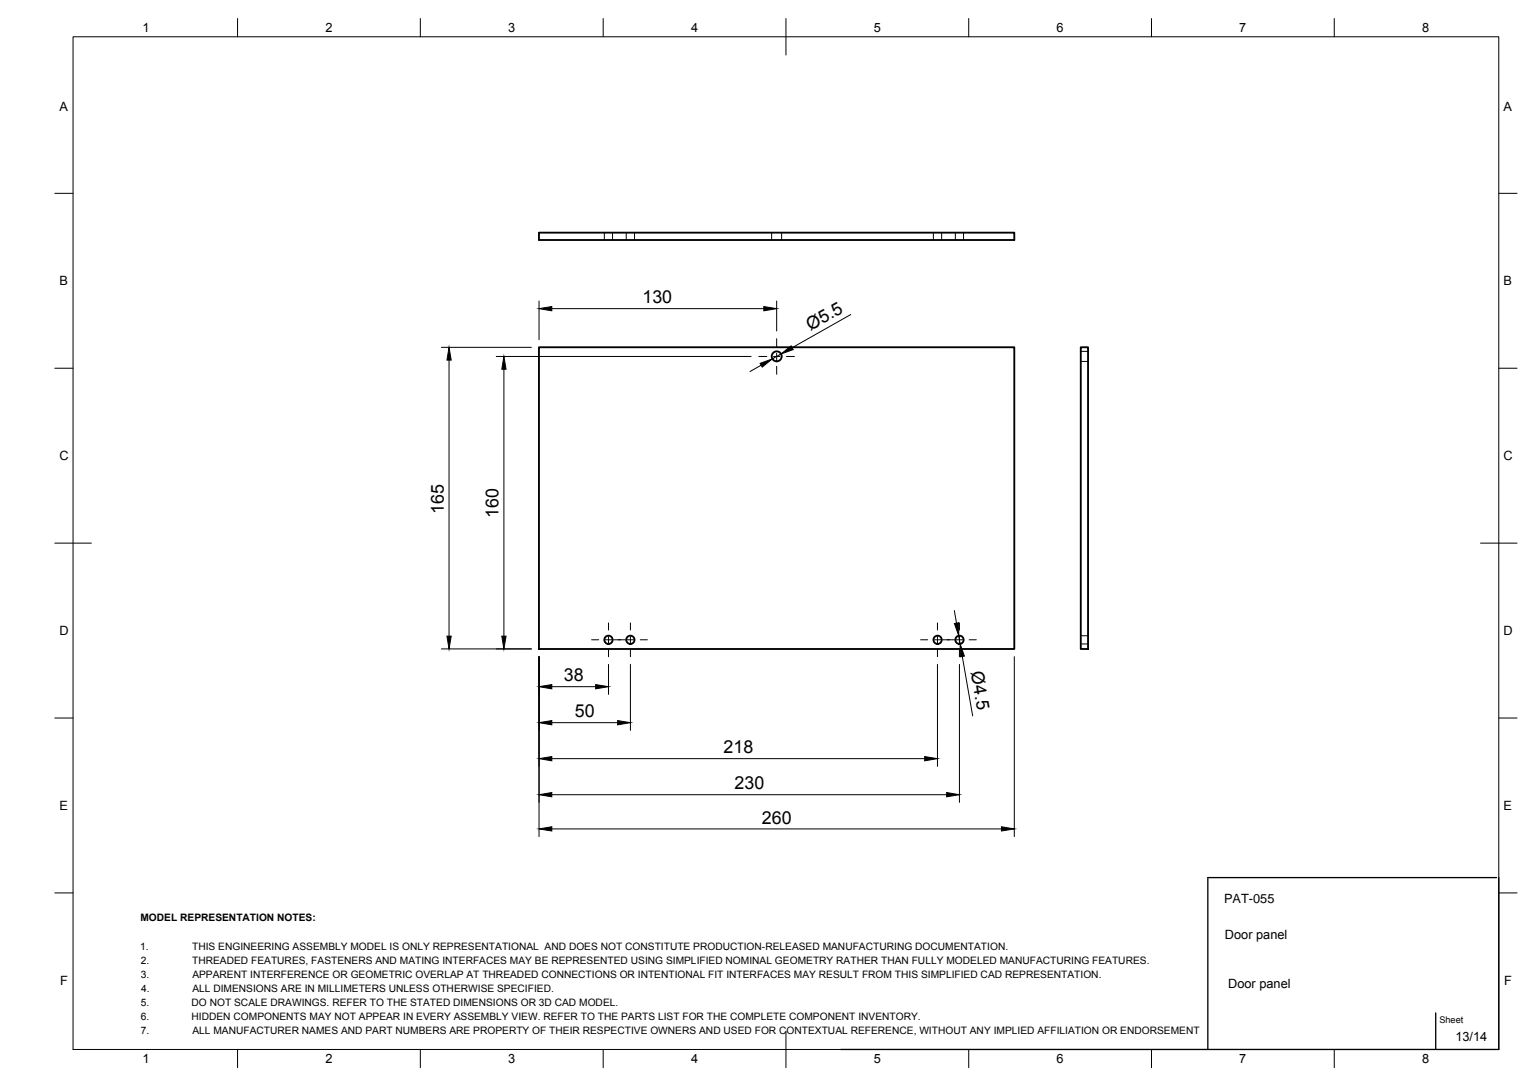
ISO-10303-21;
HEADER;
/* Generated by software containing ST-Developer
 * from STEP Tools, Inc. (www.steptools.com) 
 */

FILE_DESCRIPTION(
/* description */ ('Hinged panel with latch'),
/* implementation_level */ '2;1');

FILE_NAME(
/* name */ 'Door panel.step',
/* time_stamp */ '2026-10-27T20:36:01-07:00',
/* author */ (''),
/* organization */ (''),
/* preprocessor_version */ 'ST-DEVELOPER v20.2',
/* originating_system */ 'Autodesk Translation Framework v15.17.0.0',
/* authorisation */ '');

FILE_SCHEMA (('AUTOMOTIVE_DESIGN { 1 0 10303 214 3 1 1 }'));
ENDSEC;

DATA;
#10=MECHANICAL_DESIGN_GEOMETRIC_PRESENTATION_REPRESENTATION('',(#304),#6743);
#272=SHAPE_REPRESENTATION_RELATIONSHIP('SRR','None',#6848,#288);
#288=ADVANCED_BREP_SHAPE_REPRESENTATION('',(#319),#6734);
#304=STYLED_ITEM('',(#6989),#319);
#319=MANIFOLD_SOLID_BREP('Body1',#3807);
#346=FACE_BOUND('',#870,.T.);
#347=FACE_BOUND('',#871,.T.);
#348=FACE_BOUND('',#872,.T.);
#349=FACE_BOUND('',#873,.T.);
#350=FACE_BOUND('',#874,.T.);
#351=FACE_BOUND('',#877,.T.);
#352=FACE_BOUND('',#878,.T.);
#353=FACE_BOUND('',#879,.T.);
#354=FACE_BOUND('',#880,.T.);
#355=FACE_BOUND('',#881,.T.);
#462=PLANE('',#4181);
#463=PLANE('',#4182);
#464=PLANE('',#4183);
#465=PLANE('',#4184);
#466=PLANE('',#4185);
#467=PLANE('',#4186);
#637=FACE_OUTER_BOUND('',#864,.T.);
#638=FACE_OUTER_BOUND('',#865,.T.);
#639=FACE_OUTER_BOUND('',#866,.T.);
#640=FACE_OUTER_BOUND('',#867,.T.);
#641=FACE_OUTER_BOUND('',#868,.T.);
#642=FACE_OUTER_BOUND('',#869,.T.);
#643=FACE_OUTER_BOUND('',#875,.T.);
#644=FACE_OUTER_BOUND('',#876,.T.);
#645=FACE_OUTER_BOUND('',#882,.T.);
#646=FACE_OUTER_BOUND('',#883,.T.);
#647=FACE_OUTER_BOUND('',#884,.T.);
#864=EDGE_LOOP('',(#3162,#3163,#3164,#3165));
#865=EDGE_LOOP('',(#3166,#3167,#3168,#3169));
#866=EDGE_LOOP('',(#3170,#3171,#3172,#3173));
#867=EDGE_LOOP('',(#3174,#3175,#3176,#3177));
#868=EDGE_LOOP('',(#3178,#3179,#3180,#3181));
#869=EDGE_LOOP('',(#3182,#3183,#3184,#3185));
#870=EDGE_LOOP('',(#3186));
#871=EDGE_LOOP('',(#3187));
#872=EDGE_LOOP('',(#3188));
#873=EDGE_LOOP('',(#3189));
#874=EDGE_LOOP('',(#3190));
#875=EDGE_LOOP('',(#3191,#3192,#3193,#3194));
#876=EDGE_LOOP('',(#3195,#3196,#3197,#3198));
#877=EDGE_LOOP('',(#3199));
#878=EDGE_LOOP('',(#3200));
#879=EDGE_LOOP('',(#3201));
#880=EDGE_LOOP('',(#3202));
#881=EDGE_LOOP('',(#3203));
#882=EDGE_LOOP('',(#3204,#3205,#3206,#3207));
#883=EDGE_LOOP('',(#3208,#3209,#3210,#3211));
#884=EDGE_LOOP('',(#3212,#3213,#3214,#3215));
#1216=LINE('',#6185,#1574);
#1217=LINE('',#6191,#1575);
#1218=LINE('',#6197,#1576);
#1219=LINE('',#6203,#1577);
#1220=LINE('',#6209,#1578);
#1221=LINE('',#6214,#1579);
#1222=LINE('',#6216,#1580);
#1223=LINE('',#6218,#1581);
#1224=LINE('',#6219,#1582);
#1225=LINE('',#6222,#1583);
#1226=LINE('',#6224,#1584);
#1227=LINE('',#6225,#1585);
#1228=LINE('',#6228,#1586);
#1229=LINE('',#6230,#1587);
#1230=LINE('',#6231,#1588);
#1231=LINE('',#6233,#1589);
#1232=LINE('',#6234,#1590);
#1574=VECTOR('',#4946,0.274999999999999);
#1575=VECTOR('',#4953,0.225);
#1576=VECTOR('',#4960,0.225);
#1577=VECTOR('',#4967,0.225);
#1578=VECTOR('',#4974,0.225);
#1579=VECTOR('',#4979,1.);
#1580=VECTOR('',#4980,1.);
#1581=VECTOR('',#4981,1.);
#1582=VECTOR('',#4982,1.);
#1583=VECTOR('',#4985,1.);
#1584=VECTOR('',#4986,1.);
#1585=VECTOR('',#4987,1.);
#1586=VECTOR('',#4990,1.);
#1587=VECTOR('',#4991,1.);
#1588=VECTOR('',#4992,1.);
#1589=VECTOR('',#4995,1.);
#1590=VECTOR('',#4996,1.);
#1742=CIRCLE('',#4167,0.274999999999999);
#1743=CIRCLE('',#4168,0.274999999999999);
#1744=CIRCLE('',#4170,0.225);
#1745=CIRCLE('',#4171,0.225);
#1746=CIRCLE('',#4173,0.225);
#1747=CIRCLE('',#4174,0.225);
#1748=CIRCLE('',#4176,0.225);
#1749=CIRCLE('',#4177,0.225);
#1750=CIRCLE('',#4179,0.225);
#1751=CIRCLE('',#4180,0.225);
#1980=VERTEX_POINT('',#6182);
#1981=VERTEX_POINT('',#6184);
#1982=VERTEX_POINT('',#6188);
#1983=VERTEX_POINT('',#6190);
#1984=VERTEX_POINT('',#6194);
#1985=VERTEX_POINT('',#6196);
#1986=VERTEX_POINT('',#6200);
#1987=VERTEX_POINT('',#6202);
#1988=VERTEX_POINT('',#6206);
#1989=VERTEX_POINT('',#6208);
#1990=VERTEX_POINT('',#6212);
#1991=VERTEX_POINT('',#6213);
#1992=VERTEX_POINT('',#6215);
#1993=VERTEX_POINT('',#6217);
#1994=VERTEX_POINT('',#6221);
#1995=VERTEX_POINT('',#6223);
#1996=VERTEX_POINT('',#6227);
#1997=VERTEX_POINT('',#6229);
#2393=EDGE_CURVE('',#1980,#1980,#1742,.T.);
#2394=EDGE_CURVE('',#1980,#1981,#1216,.T.);
#2395=EDGE_CURVE('',#1981,#1981,#1743,.T.);
#2396=EDGE_CURVE('',#1982,#1982,#1744,.T.);
#2397=EDGE_CURVE('',#1982,#1983,#1217,.T.);
#2398=EDGE_CURVE('',#1983,#1983,#1745,.T.);
#2399=EDGE_CURVE('',#1984,#1984,#1746,.T.);
#2400=EDGE_CURVE('',#1984,#1985,#1218,.T.);
#2401=EDGE_CURVE('',#1985,#1985,#1747,.T.);
#2402=EDGE_CURVE('',#1986,#1986,#1748,.T.);
#2403=EDGE_CURVE('',#1986,#1987,#1219,.T.);
#2404=EDGE_CURVE('',#1987,#1987,#1749,.T.);
#2405=EDGE_CURVE('',#1988,#1988,#1750,.T.);
#2406=EDGE_CURVE('',#1988,#1989,#1220,.T.);
#2407=EDGE_CURVE('',#1989,#1989,#1751,.T.);
#2408=EDGE_CURVE('',#1990,#1991,#1221,.T.);
#2409=EDGE_CURVE('',#1991,#1992,#1222,.T.);
#2410=EDGE_CURVE('',#1993,#1992,#1223,.T.);
#2411=EDGE_CURVE('',#1990,#1993,#1224,.T.);
#2412=EDGE_CURVE('',#1994,#1990,#1225,.T.);
#2413=EDGE_CURVE('',#1995,#1993,#1226,.T.);
#2414=EDGE_CURVE('',#1994,#1995,#1227,.T.);
#2415=EDGE_CURVE('',#1996,#1994,#1228,.T.);
#2416=EDGE_CURVE('',#1997,#1995,#1229,.T.);
#2417=EDGE_CURVE('',#1996,#1997,#1230,.T.);
#2418=EDGE_CURVE('',#1991,#1996,#1231,.T.);
#2419=EDGE_CURVE('',#1992,#1997,#1232,.T.);
#3162=ORIENTED_EDGE('',*,*,#2393,.F.);
#3163=ORIENTED_EDGE('',*,*,#2394,.T.);
#3164=ORIENTED_EDGE('',*,*,#2395,.F.);
#3165=ORIENTED_EDGE('',*,*,#2394,.F.);
#3166=ORIENTED_EDGE('',*,*,#2396,.F.);
#3167=ORIENTED_EDGE('',*,*,#2397,.T.);
#3168=ORIENTED_EDGE('',*,*,#2398,.F.);
#3169=ORIENTED_EDGE('',*,*,#2397,.F.);
#3170=ORIENTED_EDGE('',*,*,#2399,.F.);
#3171=ORIENTED_EDGE('',*,*,#2400,.T.);
#3172=ORIENTED_EDGE('',*,*,#2401,.F.);
#3173=ORIENTED_EDGE('',*,*,#2400,.F.);
#3174=ORIENTED_EDGE('',*,*,#2402,.F.);
#3175=ORIENTED_EDGE('',*,*,#2403,.T.);
#3176=ORIENTED_EDGE('',*,*,#2404,.F.);
#3177=ORIENTED_EDGE('',*,*,#2403,.F.);
#3178=ORIENTED_EDGE('',*,*,#2405,.F.);
#3179=ORIENTED_EDGE('',*,*,#2406,.T.);
#3180=ORIENTED_EDGE('',*,*,#2407,.F.);
#3181=ORIENTED_EDGE('',*,*,#2406,.F.);
#3182=ORIENTED_EDGE('',*,*,#2408,.T.);
#3183=ORIENTED_EDGE('',*,*,#2409,.T.);
#3184=ORIENTED_EDGE('',*,*,#2410,.F.);
#3185=ORIENTED_EDGE('',*,*,#2411,.F.);
#3186=ORIENTED_EDGE('',*,*,#2395,.T.);
#3187=ORIENTED_EDGE('',*,*,#2398,.T.);
#3188=ORIENTED_EDGE('',*,*,#2401,.T.);
#3189=ORIENTED_EDGE('',*,*,#2404,.T.);
#3190=ORIENTED_EDGE('',*,*,#2407,.T.);
#3191=ORIENTED_EDGE('',*,*,#2412,.T.);
#3192=ORIENTED_EDGE('',*,*,#2411,.T.);
#3193=ORIENTED_EDGE('',*,*,#2413,.F.);
#3194=ORIENTED_EDGE('',*,*,#2414,.F.);
#3195=ORIENTED_EDGE('',*,*,#2415,.T.);
#3196=ORIENTED_EDGE('',*,*,#2414,.T.);
#3197=ORIENTED_EDGE('',*,*,#2416,.F.);
#3198=ORIENTED_EDGE('',*,*,#2417,.F.);
#3199=ORIENTED_EDGE('',*,*,#2393,.T.);
#3200=ORIENTED_EDGE('',*,*,#2396,.T.);
#3201=ORIENTED_EDGE('',*,*,#2399,.T.);
#3202=ORIENTED_EDGE('',*,*,#2402,.T.);
#3203=ORIENTED_EDGE('',*,*,#2405,.T.);
#3204=ORIENTED_EDGE('',*,*,#2418,.T.);
#3205=ORIENTED_EDGE('',*,*,#2417,.T.);
#3206=ORIENTED_EDGE('',*,*,#2419,.F.);
#3207=ORIENTED_EDGE('',*,*,#2409,.F.);
#3208=ORIENTED_EDGE('',*,*,#2419,.T.);
#3209=ORIENTED_EDGE('',*,*,#2416,.T.);
#3210=ORIENTED_EDGE('',*,*,#2413,.T.);
#3211=ORIENTED_EDGE('',*,*,#2410,.T.);
#3212=ORIENTED_EDGE('',*,*,#2418,.F.);
#3213=ORIENTED_EDGE('',*,*,#2408,.F.);
#3214=ORIENTED_EDGE('',*,*,#2412,.F.);
#3215=ORIENTED_EDGE('',*,*,#2415,.F.);
#3574=CYLINDRICAL_SURFACE('',#4166,0.274999999999999);
#3575=CYLINDRICAL_SURFACE('',#4169,0.225);
#3576=CYLINDRICAL_SURFACE('',#4172,0.225);
#3577=CYLINDRICAL_SURFACE('',#4175,0.225);
#3578=CYLINDRICAL_SURFACE('',#4178,0.225);
#3706=ADVANCED_FACE('',(#637),#3574,.F.);
#3707=ADVANCED_FACE('',(#638),#3575,.F.);
#3708=ADVANCED_FACE('',(#639),#3576,.F.);
#3709=ADVANCED_FACE('',(#640),#3577,.F.);
#3710=ADVANCED_FACE('',(#641),#3578,.F.);
#3711=ADVANCED_FACE('',(#642,#346,#347,#348,#349,#350),#462,.T.);
#3712=ADVANCED_FACE('',(#643),#463,.T.);
#3713=ADVANCED_FACE('',(#644,#351,#352,#353,#354,#355),#464,.T.);
#3714=ADVANCED_FACE('',(#645),#465,.T.);
#3715=ADVANCED_FACE('',(#646),#466,.T.);
#3716=ADVANCED_FACE('',(#647),#467,.F.);
#3807=CLOSED_SHELL('',(#3706,#3707,#3708,#3709,#3710,#3711,#3712,#3713,
#3714,#3715,#3716));
#4165=AXIS2_PLACEMENT_3D('',#6180,#4940,#4941);
#4166=AXIS2_PLACEMENT_3D('',#6181,#4942,#4943);
#4167=AXIS2_PLACEMENT_3D('',#6183,#4944,#4945);
#4168=AXIS2_PLACEMENT_3D('',#6186,#4947,#4948);
#4169=AXIS2_PLACEMENT_3D('',#6187,#4949,#4950);
#4170=AXIS2_PLACEMENT_3D('',#6189,#4951,#4952);
#4171=AXIS2_PLACEMENT_3D('',#6192,#4954,#4955);
#4172=AXIS2_PLACEMENT_3D('',#6193,#4956,#4957);
#4173=AXIS2_PLACEMENT_3D('',#6195,#4958,#4959);
#4174=AXIS2_PLACEMENT_3D('',#6198,#4961,#4962);
#4175=AXIS2_PLACEMENT_3D('',#6199,#4963,#4964);
#4176=AXIS2_PLACEMENT_3D('',#6201,#4965,#4966);
#4177=AXIS2_PLACEMENT_3D('',#6204,#4968,#4969);
#4178=AXIS2_PLACEMENT_3D('',#6205,#4970,#4971);
#4179=AXIS2_PLACEMENT_3D('',#6207,#4972,#4973);
#4180=AXIS2_PLACEMENT_3D('',#6210,#4975,#4976);
#4181=AXIS2_PLACEMENT_3D('',#6211,#4977,#4978);
#4182=AXIS2_PLACEMENT_3D('',#6220,#4983,#4984);
#4183=AXIS2_PLACEMENT_3D('',#6226,#4988,#4989);
#4184=AXIS2_PLACEMENT_3D('',#6232,#4993,#4994);
#4185=AXIS2_PLACEMENT_3D('',#6235,#4997,#4998);
#4186=AXIS2_PLACEMENT_3D('',#6236,#4999,#5000);
#4940=DIRECTION('axis',(0.,0.,1.));
#4941=DIRECTION('refdir',(1.,0.,0.));
#4942=DIRECTION('center_axis',(0.,1.,0.));
#4943=DIRECTION('ref_axis',(1.,0.,0.));
#4944=DIRECTION('center_axis',(0.,1.,0.));
#4945=DIRECTION('ref_axis',(1.,0.,0.));
#4946=DIRECTION('',(0.,1.,0.));
#4947=DIRECTION('center_axis',(0.,-1.,0.));
#4948=DIRECTION('ref_axis',(1.,0.,0.));
#4949=DIRECTION('center_axis',(0.,1.,0.));
#4950=DIRECTION('ref_axis',(1.,0.,0.));
#4951=DIRECTION('center_axis',(0.,1.,0.));
#4952=DIRECTION('ref_axis',(1.,0.,0.));
#4953=DIRECTION('',(0.,1.,0.));
#4954=DIRECTION('center_axis',(0.,-1.,0.));
#4955=DIRECTION('ref_axis',(1.,0.,0.));
#4956=DIRECTION('center_axis',(0.,1.,0.));
#4957=DIRECTION('ref_axis',(1.,0.,0.));
#4958=DIRECTION('center_axis',(0.,1.,0.));
#4959=DIRECTION('ref_axis',(1.,0.,0.));
#4960=DIRECTION('',(0.,1.,0.));
#4961=DIRECTION('center_axis',(0.,-1.,0.));
#4962=DIRECTION('ref_axis',(1.,0.,0.));
#4963=DIRECTION('center_axis',(0.,1.,0.));
#4964=DIRECTION('ref_axis',(1.,0.,0.));
#4965=DIRECTION('center_axis',(0.,1.,0.));
#4966=DIRECTION('ref_axis',(1.,0.,0.));
#4967=DIRECTION('',(0.,1.,0.));
#4968=DIRECTION('center_axis',(0.,-1.,0.));
#4969=DIRECTION('ref_axis',(1.,0.,0.));
#4970=DIRECTION('center_axis',(0.,1.,0.));
#4971=DIRECTION('ref_axis',(1.,0.,0.));
#4972=DIRECTION('center_axis',(0.,1.,0.));
#4973=DIRECTION('ref_axis',(1.,0.,0.));
#4974=DIRECTION('',(0.,1.,0.));
#4975=DIRECTION('center_axis',(0.,-1.,0.));
#4976=DIRECTION('ref_axis',(1.,0.,0.));
#4977=DIRECTION('center_axis',(0.,1.,0.));
#4978=DIRECTION('ref_axis',(-1.,0.,0.));
#4979=DIRECTION('',(-1.,0.,0.));
#4980=DIRECTION('',(0.,0.,1.));
#4981=DIRECTION('',(-1.,0.,0.));
#4982=DIRECTION('',(0.,0.,1.));
#4983=DIRECTION('center_axis',(1.,0.,0.));
#4984=DIRECTION('ref_axis',(0.,1.,0.));
#4985=DIRECTION('',(0.,1.,0.));
#4986=DIRECTION('',(0.,1.,0.));
#4987=DIRECTION('',(0.,0.,1.));
#4988=DIRECTION('center_axis',(0.,-1.,0.));
#4989=DIRECTION('ref_axis',(1.,0.,0.));
#4990=DIRECTION('',(1.,0.,0.));
#4991=DIRECTION('',(1.,0.,0.));
#4992=DIRECTION('',(0.,0.,1.));
#4993=DIRECTION('center_axis',(-1.,0.,0.));
#4994=DIRECTION('ref_axis',(0.,-1.,0.));
#4995=DIRECTION('',(0.,-1.,0.));
#4996=DIRECTION('',(0.,-1.,0.));
#4997=DIRECTION('center_axis',(0.,0.,1.));
#4998=DIRECTION('ref_axis',(1.,0.,0.));
#4999=DIRECTION('center_axis',(0.,0.,1.));
#5000=DIRECTION('ref_axis',(1.,0.,0.));
#6180=CARTESIAN_POINT('',(0.,0.,0.));
#6181=CARTESIAN_POINT('Origin',(20.,-1.9,16.));
#6182=CARTESIAN_POINT('',(19.725,-1.8,16.));
#6183=CARTESIAN_POINT('Origin',(20.,-1.8,16.));
#6184=CARTESIAN_POINT('',(19.725,-1.4,16.));
#6185=CARTESIAN_POINT('',(19.725,-1.9,16.));
#6186=CARTESIAN_POINT('Origin',(20.,-1.4,16.));
#6187=CARTESIAN_POINT('Origin',(4.5,-1.9,24.));
#6188=CARTESIAN_POINT('',(4.275,-1.8,24.));
#6189=CARTESIAN_POINT('Origin',(4.5,-1.8,24.));
#6190=CARTESIAN_POINT('',(4.275,-1.4,24.));
#6191=CARTESIAN_POINT('',(4.275,-1.9,24.));
#6192=CARTESIAN_POINT('Origin',(4.5,-1.4,24.));
#6193=CARTESIAN_POINT('Origin',(4.5,-1.9,7.2));
#6194=CARTESIAN_POINT('',(4.275,-1.8,7.2));
#6195=CARTESIAN_POINT('Origin',(4.5,-1.8,7.2));
#6196=CARTESIAN_POINT('',(4.275,-1.4,7.2));
#6197=CARTESIAN_POINT('',(4.275,-1.9,7.2));
#6198=CARTESIAN_POINT('Origin',(4.5,-1.4,7.2));
#6199=CARTESIAN_POINT('Origin',(4.5,-1.9,6.));
#6200=CARTESIAN_POINT('',(4.275,-1.8,6.));
#6201=CARTESIAN_POINT('Origin',(4.5,-1.8,6.));
#6202=CARTESIAN_POINT('',(4.275,-1.4,6.));
#6203=CARTESIAN_POINT('',(4.275,-1.9,6.));
#6204=CARTESIAN_POINT('Origin',(4.5,-1.4,6.));
#6205=CARTESIAN_POINT('Origin',(4.5,-1.9,25.2));
#6206=CARTESIAN_POINT('',(4.275,-1.8,25.2));
#6207=CARTESIAN_POINT('Origin',(4.5,-1.8,25.2));
#6208=CARTESIAN_POINT('',(4.275,-1.4,25.2));
#6209=CARTESIAN_POINT('',(4.275,-1.9,25.2));
#6210=CARTESIAN_POINT('Origin',(4.5,-1.4,25.2));
#6211=CARTESIAN_POINT('Origin',(20.5,-1.4,3.));
#6212=CARTESIAN_POINT('',(20.5,-1.4,3.));
#6213=CARTESIAN_POINT('',(4.,-1.4,3.));
#6214=CARTESIAN_POINT('',(20.5,-1.4,3.));
#6215=CARTESIAN_POINT('',(4.,-1.4,29.));
#6216=CARTESIAN_POINT('',(4.,-1.4,3.));
#6217=CARTESIAN_POINT('',(20.5,-1.4,29.));
#6218=CARTESIAN_POINT('',(20.5,-1.4,29.));
#6219=CARTESIAN_POINT('',(20.5,-1.4,3.));
#6220=CARTESIAN_POINT('Origin',(20.5,-1.8,3.));
#6221=CARTESIAN_POINT('',(20.5,-1.8,3.));
#6222=CARTESIAN_POINT('',(20.5,-1.8,3.));
#6223=CARTESIAN_POINT('',(20.5,-1.8,29.));
#6224=CARTESIAN_POINT('',(20.5,-1.8,29.));
#6225=CARTESIAN_POINT('',(20.5,-1.8,3.));
#6226=CARTESIAN_POINT('Origin',(4.,-1.8,3.));
#6227=CARTESIAN_POINT('',(4.,-1.8,3.));
#6228=CARTESIAN_POINT('',(4.,-1.8,3.));
#6229=CARTESIAN_POINT('',(4.,-1.8,29.));
#6230=CARTESIAN_POINT('',(4.,-1.8,29.));
#6231=CARTESIAN_POINT('',(4.,-1.8,3.));
#6232=CARTESIAN_POINT('Origin',(4.,-1.4,3.));
#6233=CARTESIAN_POINT('',(4.,-1.4,3.));
#6234=CARTESIAN_POINT('',(4.,-1.4,29.));
#6235=CARTESIAN_POINT('Origin',(12.25,-1.6,29.));
#6236=CARTESIAN_POINT('Origin',(12.25,-1.6,3.));
#6713=UNCERTAINTY_MEASURE_WITH_UNIT(LENGTH_MEASURE(0.001),#6744,
'DISTANCE_ACCURACY_VALUE',
'Maximum model space distance between geometric entities at asserted c
onnectivities');
#6722=UNCERTAINTY_MEASURE_WITH_UNIT(LENGTH_MEASURE(0.001),#6744,
'DISTANCE_ACCURACY_VALUE',
'Maximum model space distance between geometric entities at asserted c
onnectivities');
#6734=(
GEOMETRIC_REPRESENTATION_CONTEXT(3)
GLOBAL_UNCERTAINTY_ASSIGNED_CONTEXT((#6713))
GLOBAL_UNIT_ASSIGNED_CONTEXT((#6744,#6746,#6747))
REPRESENTATION_CONTEXT('','3D')
);
#6743=(
GEOMETRIC_REPRESENTATION_CONTEXT(3)
GLOBAL_UNCERTAINTY_ASSIGNED_CONTEXT((#6722))
GLOBAL_UNIT_ASSIGNED_CONTEXT((#6744,#6746,#6747))
REPRESENTATION_CONTEXT('','3D')
);
#6744=(
LENGTH_UNIT()
NAMED_UNIT(*)
SI_UNIT(.CENTI.,.METRE.)
);
#6746=(
NAMED_UNIT(*)
PLANE_ANGLE_UNIT()
SI_UNIT($,.RADIAN.)
);
#6747=(
NAMED_UNIT(*)
SI_UNIT($,.STERADIAN.)
SOLID_ANGLE_UNIT()
);
#6759=SHAPE_DEFINITION_REPRESENTATION(#6779,#6848);
#6779=PRODUCT_DEFINITION_SHAPE('',$,#6869);
#6848=SHAPE_REPRESENTATION('',(#4165),#6734);
#6857=PRODUCT_DEFINITION_CONTEXT('part definition',#6919,'design');
#6869=PRODUCT_DEFINITION('Door panel','Door panel',#6889,#6857);
#6889=PRODUCT_DEFINITION_FORMATION('',$,#6932);
#6919=APPLICATION_CONTEXT(
'Core Data for Automotive Mechanical Design Process');
#6920=PRODUCT_CONTEXT('part definition',#6919,'mechanical');
#6932=PRODUCT('Door panel','Door panel','Door panel',(#6920));
#6983=COLOUR_RGB('Light Blue',0.38,0.62,0.78);
#6984=FILL_AREA_STYLE_COLOUR('',#6983);
#6985=FILL_AREA_STYLE('',(#6984));
#6986=SURFACE_STYLE_FILL_AREA(#6985);
#6987=SURFACE_SIDE_STYLE('',(#6986));
#6988=SURFACE_STYLE_USAGE(.BOTH.,#6987);
#6989=PRESENTATION_STYLE_ASSIGNMENT((#6988));
ENDSEC;
END-ISO-10303-21;
